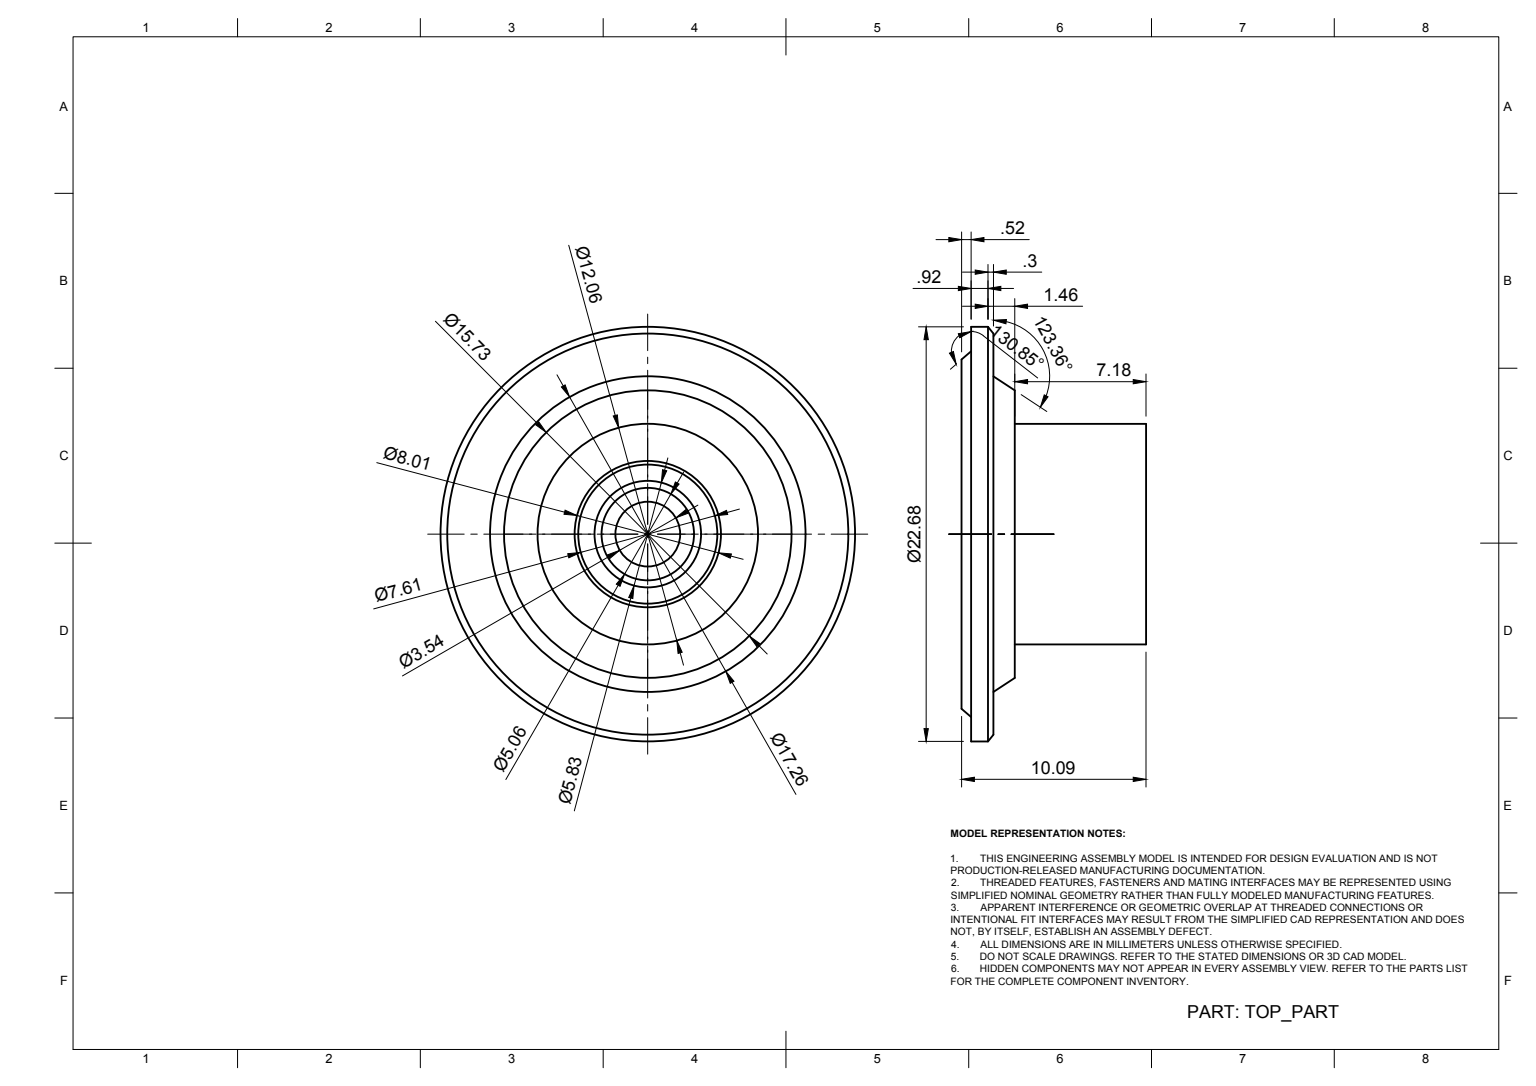
ISO-10303-21;
HEADER;
/* Generated by software containing ST-Developer
 * from STEP Tools, Inc. (www.steptools.com) 
 */

FILE_DESCRIPTION(
/* description */ (''),
/* implementation_level */ '2;1');

FILE_NAME(
/* name */ 'Top_Part.step',
/* time_stamp */ '2026-10-04T22:56:18-07:00',
/* author */ (''),
/* organization */ (''),
/* preprocessor_version */ 'ST-DEVELOPER v20.2',
/* originating_system */ 'Autodesk Translation Framework v15.15.0.0',
/* authorisation */ '');

FILE_SCHEMA (('AUTOMOTIVE_DESIGN { 1 0 10303 214 3 1 1 }'));
ENDSEC;

DATA;
#10=MECHANICAL_DESIGN_GEOMETRIC_PRESENTATION_REPRESENTATION('',(#196),#14544);
#44=CONICAL_SURFACE('',#2051,6.94221583892671,0.735432745767903);
#45=CONICAL_SURFACE('',#2055,9.77637943942299,0.712897062744303);
#46=CONICAL_SURFACE('',#2061,11.1537701181833,0.893668754257897);
#47=CONICAL_SURFACE('',#2065,8.2465180845384,0.582247271411204);
#48=CONICAL_SURFACE('',#2073,3.90337928524842,0.252845151189765);
#49=CONICAL_SURFACE('',#2083,2.14952775522097,1.03539162387167);
#180=SHAPE_REPRESENTATION_RELATIONSHIP('SRR','None',#14582,#188);
#188=ADVANCED_BREP_SHAPE_REPRESENTATION('',(#204),#14542);
#196=STYLED_ITEM('',(#14627),#204);
#204=MANIFOLD_SOLID_BREP('Body1',#1832);
#240=LINE('',#8609,#296);
#241=LINE('',#8617,#297);
#242=LINE('',#8624,#298);
#243=LINE('',#8627,#299);
#244=LINE('',#8634,#300);
#245=LINE('',#8642,#301);
#246=LINE('',#8649,#302);
#247=LINE('',#8656,#303);
#248=LINE('',#8663,#304);
#249=LINE('',#8667,#305);
#250=LINE('',#8669,#306);
#296=VECTOR('',#2420,6.94221583892671);
#297=VECTOR('',#2431,9.77637943942299);
#298=VECTOR('',#2440,11.3384150169577);
#299=VECTOR('',#2443,11.1537701181833);
#300=VECTOR('',#2452,8.2465180845384);
#301=VECTOR('',#2463,6.03157539652109);
#302=VECTOR('',#2472,3.90337928524842);
#303=VECTOR('',#2481,2.91473371720024);
#304=VECTOR('',#2490,2.52802020062926);
#305=VECTOR('',#2495,2.14952775522097);
#306=VECTOR('',#2498,1.77103530981268);
#353=CYLINDRICAL_SURFACE('',#2059,11.3384150169577);
#354=CYLINDRICAL_SURFACE('',#2069,6.03157539652109);
#355=CYLINDRICAL_SURFACE('',#2077,2.91473371720024);
#356=CYLINDRICAL_SURFACE('',#2081,2.52802020062926);
#357=CYLINDRICAL_SURFACE('',#2085,1.77103530981268);
#389=FACE_BOUND('',#589,.T.);
#390=FACE_BOUND('',#592,.T.);
#391=FACE_BOUND('',#595,.T.);
#392=FACE_BOUND('',#599,.T.);
#393=FACE_BOUND('',#602,.T.);
#394=FACE_BOUND('',#605,.T.);
#395=FACE_BOUND('',#608,.T.);
#396=FACE_BOUND('',#611,.T.);
#464=FACE_OUTER_BOUND('',#588,.T.);
#465=FACE_OUTER_BOUND('',#590,.T.);
#466=FACE_OUTER_BOUND('',#591,.T.);
#467=FACE_OUTER_BOUND('',#593,.T.);
#468=FACE_OUTER_BOUND('',#594,.T.);
#469=FACE_OUTER_BOUND('',#596,.T.);
#470=FACE_OUTER_BOUND('',#597,.T.);
#471=FACE_OUTER_BOUND('',#598,.T.);
#472=FACE_OUTER_BOUND('',#600,.T.);
#473=FACE_OUTER_BOUND('',#601,.T.);
#474=FACE_OUTER_BOUND('',#603,.T.);
#475=FACE_OUTER_BOUND('',#604,.T.);
#476=FACE_OUTER_BOUND('',#606,.T.);
#477=FACE_OUTER_BOUND('',#607,.T.);
#478=FACE_OUTER_BOUND('',#609,.T.);
#479=FACE_OUTER_BOUND('',#610,.T.);
#480=FACE_OUTER_BOUND('',#612,.T.);
#481=FACE_OUTER_BOUND('',#613,.T.);
#482=FACE_OUTER_BOUND('',#614,.T.);
#588=EDGE_LOOP('',(#1481));
#589=EDGE_LOOP('',(#1482));
#590=EDGE_LOOP('',(#1483,#1484,#1485,#1486));
#591=EDGE_LOOP('',(#1487));
#592=EDGE_LOOP('',(#1488));
#593=EDGE_LOOP('',(#1489,#1490,#1491,#1492));
#594=EDGE_LOOP('',(#1493));
#595=EDGE_LOOP('',(#1494));
#596=EDGE_LOOP('',(#1495,#1496,#1497,#1498));
#597=EDGE_LOOP('',(#1499,#1500,#1501,#1502));
#598=EDGE_LOOP('',(#1503));
#599=EDGE_LOOP('',(#1504));
#600=EDGE_LOOP('',(#1505,#1506,#1507,#1508));
#601=EDGE_LOOP('',(#1509));
#602=EDGE_LOOP('',(#1510));
#603=EDGE_LOOP('',(#1511,#1512,#1513,#1514));
#604=EDGE_LOOP('',(#1515));
#605=EDGE_LOOP('',(#1516));
#606=EDGE_LOOP('',(#1517,#1518,#1519,#1520));
#607=EDGE_LOOP('',(#1521));
#608=EDGE_LOOP('',(#1522));
#609=EDGE_LOOP('',(#1523,#1524,#1525,#1526));
#610=EDGE_LOOP('',(#1527));
#611=EDGE_LOOP('',(#1528));
#612=EDGE_LOOP('',(#1529,#1530,#1531,#1532));
#613=EDGE_LOOP('',(#1533,#1534,#1535,#1536));
#614=EDGE_LOOP('',(#1537,#1538,#1539,#1540));
#692=CIRCLE('',#2049,6.73223109314486);
#693=CIRCLE('',#2050,1.77103530981268);
#694=CIRCLE('',#2052,7.15220058470855);
#695=CIRCLE('',#2054,9.55065635544564);
#696=CIRCLE('',#2056,10.0021025234003);
#697=CIRCLE('',#2058,11.3384150169577);
#698=CIRCLE('',#2060,11.3384150169577);
#699=CIRCLE('',#2062,10.9691252194088);
#700=CIRCLE('',#2064,8.63028983493237);
#701=CIRCLE('',#2066,7.86274633414444);
#702=CIRCLE('',#2068,6.03157539652109);
#703=CIRCLE('',#2070,6.03157539652109);
#704=CIRCLE('',#2072,4.0030788546633);
#705=CIRCLE('',#2074,3.80367971583355);
#706=CIRCLE('',#2076,2.91473371720024);
#707=CIRCLE('',#2078,2.91473371720024);
#708=CIRCLE('',#2080,2.52802020062926);
#709=CIRCLE('',#2082,2.52802020062926);
#710=CIRCLE('',#2084,1.77103530981268);
#840=VERTEX_POINT('',#8603);
#841=VERTEX_POINT('',#8605);
#842=VERTEX_POINT('',#8608);
#843=VERTEX_POINT('',#8612);
#844=VERTEX_POINT('',#8615);
#845=VERTEX_POINT('',#8619);
#846=VERTEX_POINT('',#8622);
#847=VERTEX_POINT('',#8626);
#848=VERTEX_POINT('',#8630);
#849=VERTEX_POINT('',#8633);
#850=VERTEX_POINT('',#8637);
#851=VERTEX_POINT('',#8640);
#852=VERTEX_POINT('',#8644);
#853=VERTEX_POINT('',#8647);
#854=VERTEX_POINT('',#8651);
#855=VERTEX_POINT('',#8654);
#856=VERTEX_POINT('',#8658);
#857=VERTEX_POINT('',#8661);
#858=VERTEX_POINT('',#8665);
#1069=EDGE_CURVE('',#840,#840,#692,.T.);
#1070=EDGE_CURVE('',#841,#841,#693,.T.);
#1071=EDGE_CURVE('',#840,#842,#240,.T.);
#1072=EDGE_CURVE('',#842,#842,#694,.T.);
#1073=EDGE_CURVE('',#843,#843,#695,.T.);
#1074=EDGE_CURVE('',#844,#844,#696,.T.);
#1075=EDGE_CURVE('',#844,#843,#241,.T.);
#1076=EDGE_CURVE('',#845,#845,#697,.T.);
#1077=EDGE_CURVE('',#846,#846,#698,.T.);
#1078=EDGE_CURVE('',#846,#845,#242,.T.);
#1079=EDGE_CURVE('',#846,#847,#243,.T.);
#1080=EDGE_CURVE('',#847,#847,#699,.T.);
#1081=EDGE_CURVE('',#848,#848,#700,.T.);
#1082=EDGE_CURVE('',#848,#849,#244,.T.);
#1083=EDGE_CURVE('',#849,#849,#701,.T.);
#1084=EDGE_CURVE('',#850,#850,#702,.T.);
#1085=EDGE_CURVE('',#851,#851,#703,.T.);
#1086=EDGE_CURVE('',#851,#850,#245,.T.);
#1087=EDGE_CURVE('',#852,#852,#704,.T.);
#1088=EDGE_CURVE('',#853,#853,#705,.T.);
#1089=EDGE_CURVE('',#853,#852,#246,.T.);
#1090=EDGE_CURVE('',#854,#854,#706,.T.);
#1091=EDGE_CURVE('',#855,#855,#707,.T.);
#1092=EDGE_CURVE('',#855,#854,#247,.T.);
#1093=EDGE_CURVE('',#856,#856,#708,.T.);
#1094=EDGE_CURVE('',#857,#857,#709,.T.);
#1095=EDGE_CURVE('',#857,#856,#248,.T.);
#1096=EDGE_CURVE('',#858,#858,#710,.T.);
#1097=EDGE_CURVE('',#858,#857,#249,.T.);
#1098=EDGE_CURVE('',#841,#858,#250,.T.);
#1481=ORIENTED_EDGE('',*,*,#1069,.F.);
#1482=ORIENTED_EDGE('',*,*,#1070,.T.);
#1483=ORIENTED_EDGE('',*,*,#1069,.T.);
#1484=ORIENTED_EDGE('',*,*,#1071,.T.);
#1485=ORIENTED_EDGE('',*,*,#1072,.F.);
#1486=ORIENTED_EDGE('',*,*,#1071,.F.);
#1487=ORIENTED_EDGE('',*,*,#1073,.F.);
#1488=ORIENTED_EDGE('',*,*,#1072,.T.);
#1489=ORIENTED_EDGE('',*,*,#1074,.F.);
#1490=ORIENTED_EDGE('',*,*,#1075,.T.);
#1491=ORIENTED_EDGE('',*,*,#1073,.T.);
#1492=ORIENTED_EDGE('',*,*,#1075,.F.);
#1493=ORIENTED_EDGE('',*,*,#1076,.F.);
#1494=ORIENTED_EDGE('',*,*,#1074,.T.);
#1495=ORIENTED_EDGE('',*,*,#1077,.F.);
#1496=ORIENTED_EDGE('',*,*,#1078,.T.);
#1497=ORIENTED_EDGE('',*,*,#1076,.T.);
#1498=ORIENTED_EDGE('',*,*,#1078,.F.);
#1499=ORIENTED_EDGE('',*,*,#1077,.T.);
#1500=ORIENTED_EDGE('',*,*,#1079,.T.);
#1501=ORIENTED_EDGE('',*,*,#1080,.F.);
#1502=ORIENTED_EDGE('',*,*,#1079,.F.);
#1503=ORIENTED_EDGE('',*,*,#1080,.T.);
#1504=ORIENTED_EDGE('',*,*,#1081,.F.);
#1505=ORIENTED_EDGE('',*,*,#1081,.T.);
#1506=ORIENTED_EDGE('',*,*,#1082,.T.);
#1507=ORIENTED_EDGE('',*,*,#1083,.F.);
#1508=ORIENTED_EDGE('',*,*,#1082,.F.);
#1509=ORIENTED_EDGE('',*,*,#1083,.T.);
#1510=ORIENTED_EDGE('',*,*,#1084,.F.);
#1511=ORIENTED_EDGE('',*,*,#1085,.F.);
#1512=ORIENTED_EDGE('',*,*,#1086,.T.);
#1513=ORIENTED_EDGE('',*,*,#1084,.T.);
#1514=ORIENTED_EDGE('',*,*,#1086,.F.);
#1515=ORIENTED_EDGE('',*,*,#1085,.T.);
#1516=ORIENTED_EDGE('',*,*,#1087,.F.);
#1517=ORIENTED_EDGE('',*,*,#1088,.F.);
#1518=ORIENTED_EDGE('',*,*,#1089,.T.);
#1519=ORIENTED_EDGE('',*,*,#1087,.T.);
#1520=ORIENTED_EDGE('',*,*,#1089,.F.);
#1521=ORIENTED_EDGE('',*,*,#1088,.T.);
#1522=ORIENTED_EDGE('',*,*,#1090,.F.);
#1523=ORIENTED_EDGE('',*,*,#1091,.F.);
#1524=ORIENTED_EDGE('',*,*,#1092,.T.);
#1525=ORIENTED_EDGE('',*,*,#1090,.T.);
#1526=ORIENTED_EDGE('',*,*,#1092,.F.);
#1527=ORIENTED_EDGE('',*,*,#1091,.T.);
#1528=ORIENTED_EDGE('',*,*,#1093,.F.);
#1529=ORIENTED_EDGE('',*,*,#1094,.F.);
#1530=ORIENTED_EDGE('',*,*,#1095,.T.);
#1531=ORIENTED_EDGE('',*,*,#1093,.T.);
#1532=ORIENTED_EDGE('',*,*,#1095,.F.);
#1533=ORIENTED_EDGE('',*,*,#1096,.F.);
#1534=ORIENTED_EDGE('',*,*,#1097,.T.);
#1535=ORIENTED_EDGE('',*,*,#1094,.T.);
#1536=ORIENTED_EDGE('',*,*,#1097,.F.);
#1537=ORIENTED_EDGE('',*,*,#1070,.F.);
#1538=ORIENTED_EDGE('',*,*,#1098,.T.);
#1539=ORIENTED_EDGE('',*,*,#1096,.T.);
#1540=ORIENTED_EDGE('',*,*,#1098,.F.);
#1708=PLANE('',#2048);
#1709=PLANE('',#2053);
#1710=PLANE('',#2057);
#1711=PLANE('',#2063);
#1712=PLANE('',#2067);
#1713=PLANE('',#2071);
#1714=PLANE('',#2075);
#1715=PLANE('',#2079);
#1786=ADVANCED_FACE('',(#464,#389),#1708,.T.);
#1787=ADVANCED_FACE('',(#465),#44,.F.);
#1788=ADVANCED_FACE('',(#466,#390),#1709,.T.);
#1789=ADVANCED_FACE('',(#467),#45,.T.);
#1790=ADVANCED_FACE('',(#468,#391),#1710,.T.);
#1791=ADVANCED_FACE('',(#469),#353,.T.);
#1792=ADVANCED_FACE('',(#470),#46,.T.);
#1793=ADVANCED_FACE('',(#471,#392),#1711,.T.);
#1794=ADVANCED_FACE('',(#472),#47,.T.);
#1795=ADVANCED_FACE('',(#473,#393),#1712,.T.);
#1796=ADVANCED_FACE('',(#474),#354,.T.);
#1797=ADVANCED_FACE('',(#475,#394),#1713,.T.);
#1798=ADVANCED_FACE('',(#476),#48,.F.);
#1799=ADVANCED_FACE('',(#477,#395),#1714,.T.);
#1800=ADVANCED_FACE('',(#478),#355,.F.);
#1801=ADVANCED_FACE('',(#479,#396),#1715,.T.);
#1802=ADVANCED_FACE('',(#480),#356,.F.);
#1803=ADVANCED_FACE('',(#481),#49,.F.);
#1804=ADVANCED_FACE('',(#482),#357,.F.);
#1832=CLOSED_SHELL('',(#1786,#1787,#1788,#1789,#1790,#1791,#1792,#1793,
#1794,#1795,#1796,#1797,#1798,#1799,#1800,#1801,#1802,#1803,#1804));
#2047=AXIS2_PLACEMENT_3D('',#8601,#2410,#2411);
#2048=AXIS2_PLACEMENT_3D('',#8602,#2412,#2413);
#2049=AXIS2_PLACEMENT_3D('',#8604,#2414,#2415);
#2050=AXIS2_PLACEMENT_3D('',#8606,#2416,#2417);
#2051=AXIS2_PLACEMENT_3D('',#8607,#2418,#2419);
#2052=AXIS2_PLACEMENT_3D('',#8610,#2421,#2422);
#2053=AXIS2_PLACEMENT_3D('',#8611,#2423,#2424);
#2054=AXIS2_PLACEMENT_3D('',#8613,#2425,#2426);
#2055=AXIS2_PLACEMENT_3D('',#8614,#2427,#2428);
#2056=AXIS2_PLACEMENT_3D('',#8616,#2429,#2430);
#2057=AXIS2_PLACEMENT_3D('',#8618,#2432,#2433);
#2058=AXIS2_PLACEMENT_3D('',#8620,#2434,#2435);
#2059=AXIS2_PLACEMENT_3D('',#8621,#2436,#2437);
#2060=AXIS2_PLACEMENT_3D('',#8623,#2438,#2439);
#2061=AXIS2_PLACEMENT_3D('',#8625,#2441,#2442);
#2062=AXIS2_PLACEMENT_3D('',#8628,#2444,#2445);
#2063=AXIS2_PLACEMENT_3D('',#8629,#2446,#2447);
#2064=AXIS2_PLACEMENT_3D('',#8631,#2448,#2449);
#2065=AXIS2_PLACEMENT_3D('',#8632,#2450,#2451);
#2066=AXIS2_PLACEMENT_3D('',#8635,#2453,#2454);
#2067=AXIS2_PLACEMENT_3D('',#8636,#2455,#2456);
#2068=AXIS2_PLACEMENT_3D('',#8638,#2457,#2458);
#2069=AXIS2_PLACEMENT_3D('',#8639,#2459,#2460);
#2070=AXIS2_PLACEMENT_3D('',#8641,#2461,#2462);
#2071=AXIS2_PLACEMENT_3D('',#8643,#2464,#2465);
#2072=AXIS2_PLACEMENT_3D('',#8645,#2466,#2467);
#2073=AXIS2_PLACEMENT_3D('',#8646,#2468,#2469);
#2074=AXIS2_PLACEMENT_3D('',#8648,#2470,#2471);
#2075=AXIS2_PLACEMENT_3D('',#8650,#2473,#2474);
#2076=AXIS2_PLACEMENT_3D('',#8652,#2475,#2476);
#2077=AXIS2_PLACEMENT_3D('',#8653,#2477,#2478);
#2078=AXIS2_PLACEMENT_3D('',#8655,#2479,#2480);
#2079=AXIS2_PLACEMENT_3D('',#8657,#2482,#2483);
#2080=AXIS2_PLACEMENT_3D('',#8659,#2484,#2485);
#2081=AXIS2_PLACEMENT_3D('',#8660,#2486,#2487);
#2082=AXIS2_PLACEMENT_3D('',#8662,#2488,#2489);
#2083=AXIS2_PLACEMENT_3D('',#8664,#2491,#2492);
#2084=AXIS2_PLACEMENT_3D('',#8666,#2493,#2494);
#2085=AXIS2_PLACEMENT_3D('',#8668,#2496,#2497);
#2410=DIRECTION('axis',(0.,0.,1.));
#2411=DIRECTION('refdir',(1.,0.,0.));
#2412=DIRECTION('center_axis',(0.,0.,-1.));
#2413=DIRECTION('ref_axis',(-1.,0.,0.));
#2414=DIRECTION('center_axis',(0.,0.,1.));
#2415=DIRECTION('ref_axis',(1.,0.,0.));
#2416=DIRECTION('center_axis',(0.,0.,1.));
#2417=DIRECTION('ref_axis',(1.,0.,0.));
#2418=DIRECTION('center_axis',(0.,0.,-1.));
#2419=DIRECTION('ref_axis',(1.,0.,0.));
#2420=DIRECTION('',(-0.670908116956861,8.21625477953198E-17,-0.74154049019686));
#2421=DIRECTION('center_axis',(0.,0.,1.));
#2422=DIRECTION('ref_axis',(1.,0.,0.));
#2423=DIRECTION('center_axis',(0.,0.,-1.));
#2424=DIRECTION('ref_axis',(-1.,0.,0.));
#2425=DIRECTION('center_axis',(0.,0.,1.));
#2426=DIRECTION('ref_axis',(1.,0.,0.));
#2427=DIRECTION('center_axis',(0.,0.,1.));
#2428=DIRECTION('ref_axis',(1.,0.,0.));
#2429=DIRECTION('center_axis',(0.,0.,1.));
#2430=DIRECTION('ref_axis',(1.,0.,0.));
#2431=DIRECTION('',(0.654028054476354,8.00953363467037E-17,-0.756470292845579));
#2432=DIRECTION('center_axis',(0.,0.,-1.));
#2433=DIRECTION('ref_axis',(-1.,0.,0.));
#2434=DIRECTION('center_axis',(0.,0.,1.));
#2435=DIRECTION('ref_axis',(1.,0.,0.));
#2436=DIRECTION('center_axis',(0.,0.,1.));
#2437=DIRECTION('ref_axis',(1.,0.,0.));
#2438=DIRECTION('center_axis',(0.,0.,1.));
#2439=DIRECTION('ref_axis',(1.,0.,0.));
#2440=DIRECTION('',(0.,0.,-1.));
#2441=DIRECTION('center_axis',(0.,0.,-1.));
#2442=DIRECTION('ref_axis',(1.,0.,0.));
#2443=DIRECTION('',(0.77937567080628,-9.54459920586232E-17,0.626556911824666));
#2444=DIRECTION('center_axis',(0.,0.,1.));
#2445=DIRECTION('ref_axis',(1.,0.,0.));
#2446=DIRECTION('center_axis',(0.,0.,1.));
#2447=DIRECTION('ref_axis',(1.,0.,0.));
#2448=DIRECTION('center_axis',(0.,0.,1.));
#2449=DIRECTION('ref_axis',(1.,0.,0.));
#2450=DIRECTION('center_axis',(0.,0.,-1.));
#2451=DIRECTION('ref_axis',(1.,0.,0.));
#2452=DIRECTION('',(0.549902309986816,-6.7343610376909E-17,0.835228980262996));
#2453=DIRECTION('center_axis',(0.,0.,1.));
#2454=DIRECTION('ref_axis',(1.,0.,0.));
#2455=DIRECTION('center_axis',(0.,0.,1.));
#2456=DIRECTION('ref_axis',(1.,0.,0.));
#2457=DIRECTION('center_axis',(0.,0.,1.));
#2458=DIRECTION('ref_axis',(1.,0.,0.));
#2459=DIRECTION('center_axis',(0.,0.,1.));
#2460=DIRECTION('ref_axis',(1.,0.,0.));
#2461=DIRECTION('center_axis',(0.,0.,1.));
#2462=DIRECTION('ref_axis',(1.,0.,0.));
#2463=DIRECTION('',(0.,0.,-1.));
#2464=DIRECTION('center_axis',(0.,0.,1.));
#2465=DIRECTION('ref_axis',(1.,0.,0.));
#2466=DIRECTION('center_axis',(0.,0.,1.));
#2467=DIRECTION('ref_axis',(1.,0.,0.));
#2468=DIRECTION('center_axis',(0.,0.,1.));
#2469=DIRECTION('ref_axis',(1.,0.,0.));
#2470=DIRECTION('center_axis',(0.,0.,1.));
#2471=DIRECTION('ref_axis',(1.,0.,0.));
#2472=DIRECTION('',(-0.250159656512074,-3.06357222623313E-17,0.968204599376475));
#2473=DIRECTION('center_axis',(0.,0.,1.));
#2474=DIRECTION('ref_axis',(1.,0.,0.));
#2475=DIRECTION('center_axis',(0.,0.,1.));
#2476=DIRECTION('ref_axis',(1.,0.,0.));
#2477=DIRECTION('center_axis',(0.,0.,1.));
#2478=DIRECTION('ref_axis',(1.,0.,0.));
#2479=DIRECTION('center_axis',(0.,0.,1.));
#2480=DIRECTION('ref_axis',(1.,0.,0.));
#2481=DIRECTION('',(0.,0.,1.));
#2482=DIRECTION('center_axis',(0.,0.,1.));
#2483=DIRECTION('ref_axis',(1.,0.,0.));
#2484=DIRECTION('center_axis',(0.,0.,1.));
#2485=DIRECTION('ref_axis',(1.,0.,0.));
#2486=DIRECTION('center_axis',(0.,0.,1.));
#2487=DIRECTION('ref_axis',(1.,0.,0.));
#2488=DIRECTION('center_axis',(0.,0.,1.));
#2489=DIRECTION('ref_axis',(1.,0.,0.));
#2490=DIRECTION('',(0.,0.,1.));
#2491=DIRECTION('center_axis',(0.,0.,1.));
#2492=DIRECTION('ref_axis',(1.,0.,0.));
#2493=DIRECTION('center_axis',(0.,0.,1.));
#2494=DIRECTION('ref_axis',(1.,0.,0.));
#2495=DIRECTION('',(-0.860062224672037,-1.05327245051216E-16,0.510189150896202));
#2496=DIRECTION('center_axis',(0.,0.,1.));
#2497=DIRECTION('ref_axis',(1.,0.,0.));
#2498=DIRECTION('',(0.,0.,1.));
#8601=CARTESIAN_POINT('',(0.,0.,0.));
#8602=CARTESIAN_POINT('Origin',(6.73223109314486,0.,86.2971179986903));
#8603=CARTESIAN_POINT('',(-6.73223109314486,-8.24460525934014E-16,86.2971179986903));
#8604=CARTESIAN_POINT('Origin',(0.,0.,86.2971179986903));
#8605=CARTESIAN_POINT('',(-1.77103530981268,-2.16889272333904E-16,86.2971179986903));
#8606=CARTESIAN_POINT('Origin',(0.,0.,86.2971179986903));
#8607=CARTESIAN_POINT('Origin',(0.,0.,86.0650263196877));
#8608=CARTESIAN_POINT('',(-7.15220058470855,-8.75891955292316E-16,85.8329346406852));
#8609=CARTESIAN_POINT('',(-6.94221583892671,8.50176240613165E-16,86.0650263196877));
#8610=CARTESIAN_POINT('Origin',(0.,0.,85.8329346406852));
#8611=CARTESIAN_POINT('Origin',(9.55065635544564,0.,85.8329346406852));
#8612=CARTESIAN_POINT('',(-9.55065635544564,-1.16961807354528E-15,85.8329346406852));
#8613=CARTESIAN_POINT('Origin',(0.,0.,85.8329346406852));
#8614=CARTESIAN_POINT('Origin',(0.,0.,86.0940133608864));
#8615=CARTESIAN_POINT('',(-10.0021025234003,-1.22490428400259E-15,86.3550920810876));
#8616=CARTESIAN_POINT('Origin',(0.,0.,86.3550920810876));
#8617=CARTESIAN_POINT('',(-9.77637943942299,-1.19726117877394E-15,86.0940133608864));
#8618=CARTESIAN_POINT('Origin',(11.3384150169577,0.,86.3550920810876));
#8619=CARTESIAN_POINT('',(-11.3384150169577,-1.38855536579215E-15,86.3550920810876));
#8620=CARTESIAN_POINT('Origin',(0.,0.,86.3550920810876));
#8621=CARTESIAN_POINT('Origin',(0.,0.,86.8168854949443));
#8622=CARTESIAN_POINT('',(-11.3384150169577,-1.38855536579215E-15,87.278678908801));
#8623=CARTESIAN_POINT('Origin',(0.,0.,87.278678908801));
#8624=CARTESIAN_POINT('',(-11.3384150169577,-1.38855536579215E-15,86.8168854949443));
#8625=CARTESIAN_POINT('Origin',(0.,0.,87.4271189254628));
#8626=CARTESIAN_POINT('',(-10.9691252194088,-1.34333040893955E-15,87.5755589421246));
#8627=CARTESIAN_POINT('',(-11.1537701181833,1.36594288736586E-15,87.4271189254628));
#8628=CARTESIAN_POINT('Origin',(0.,0.,87.5755589421246));
#8629=CARTESIAN_POINT('Origin',(8.63028983493237,0.,87.5755589421246));
#8630=CARTESIAN_POINT('',(-8.63028983493237,-1.05690568220639E-15,87.5755589421246));
#8631=CARTESIAN_POINT('Origin',(0.,0.,87.5755589421246));
#8632=CARTESIAN_POINT('Origin',(0.,0.,88.1584575441381));
#8633=CARTESIAN_POINT('',(-7.86274633414444,-9.62908713061757E-16,88.7413561461516));
#8634=CARTESIAN_POINT('',(-8.2465180845384,1.00990719763407E-15,88.1584575441381));
#8635=CARTESIAN_POINT('Origin',(0.,0.,88.7413561461516));
#8636=CARTESIAN_POINT('Origin',(6.03157539652109,0.,88.7413561461516));
#8637=CARTESIAN_POINT('',(-6.03157539652109,-7.38654950316548E-16,88.7413561461516));
#8638=CARTESIAN_POINT('Origin',(0.,0.,88.7413561461516));
#8639=CARTESIAN_POINT('Origin',(0.,0.,92.3318522386825));
#8640=CARTESIAN_POINT('',(-6.03157539652109,-7.38654950316548E-16,95.9223483312135));
#8641=CARTESIAN_POINT('Origin',(0.,0.,95.9223483312135));
#8642=CARTESIAN_POINT('',(-6.03157539652109,-7.38654950316548E-16,92.3318522386825));
#8643=CARTESIAN_POINT('Origin',(4.0030788546633,0.,95.9223483312135));
#8644=CARTESIAN_POINT('',(-4.0030788546633,-4.90235770609787E-16,95.9223483312135));
#8645=CARTESIAN_POINT('Origin',(0.,0.,95.9223483312135));
#8646=CARTESIAN_POINT('Origin',(0.,0.,95.536476432406));
#8647=CARTESIAN_POINT('',(-3.80367971583355,-4.65816418897727E-16,95.1506045335986));
#8648=CARTESIAN_POINT('Origin',(0.,0.,95.1506045335986));
#8649=CARTESIAN_POINT('',(-3.90337928524842,-4.78026094753756E-16,95.536476432406));
#8650=CARTESIAN_POINT('Origin',(2.91473371720024,0.,95.1506045335986));
#8651=CARTESIAN_POINT('',(-2.91473371720024,-3.56951931713614E-16,95.1506045335986));
#8652=CARTESIAN_POINT('Origin',(0.,0.,95.1506045335986));
#8653=CARTESIAN_POINT('Origin',(0.,0.,93.4125396072643));
#8654=CARTESIAN_POINT('',(-2.91473371720024,-3.56951931713614E-16,91.6744746809301));
#8655=CARTESIAN_POINT('Origin',(0.,0.,91.6744746809301));
#8656=CARTESIAN_POINT('',(-2.91473371720024,-3.56951931713614E-16,93.4125396072643));
#8657=CARTESIAN_POINT('Origin',(2.52802020062926,0.,91.6744746809301));
#8658=CARTESIAN_POINT('',(-2.52802020062926,-3.09593184688047E-16,91.6744746809301));
#8659=CARTESIAN_POINT('Origin',(0.,0.,91.6744746809301));
#8660=CARTESIAN_POINT('Origin',(0.,0.,90.2007950732064));
#8661=CARTESIAN_POINT('',(-2.52802020062926,-3.09593184688047E-16,88.7271154654827));
#8662=CARTESIAN_POINT('Origin',(0.,0.,88.7271154654827));
#8663=CARTESIAN_POINT('',(-2.52802020062926,-3.09593184688047E-16,90.2007950732064));
#8664=CARTESIAN_POINT('Origin',(0.,0.,88.5025936415912));
#8665=CARTESIAN_POINT('',(-1.77103530981268,-2.16889272333904E-16,88.2780718176998));
#8666=CARTESIAN_POINT('Origin',(0.,0.,88.2780718176998));
#8667=CARTESIAN_POINT('',(-2.14952775522097,-2.63241228510976E-16,88.5025936415912));
#8668=CARTESIAN_POINT('Origin',(0.,0.,87.287594908195));
#8669=CARTESIAN_POINT('',(-1.77103530981268,-2.16889272333904E-16,87.287594908195));
#14532=UNCERTAINTY_MEASURE_WITH_UNIT(LENGTH_MEASURE(0.01),#14545,
'DISTANCE_ACCURACY_VALUE',
'Maximum model space distance between geometric entities at asserted c
onnectivities');
#14534=UNCERTAINTY_MEASURE_WITH_UNIT(LENGTH_MEASURE(0.01),#14545,
'DISTANCE_ACCURACY_VALUE',
'Maximum model space distance between geometric entities at asserted c
onnectivities');
#14542=(
GEOMETRIC_REPRESENTATION_CONTEXT(3)
GLOBAL_UNCERTAINTY_ASSIGNED_CONTEXT((#14532))
GLOBAL_UNIT_ASSIGNED_CONTEXT((#14545,#14547,#14548))
REPRESENTATION_CONTEXT('','3D')
);
#14544=(
GEOMETRIC_REPRESENTATION_CONTEXT(3)
GLOBAL_UNCERTAINTY_ASSIGNED_CONTEXT((#14534))
GLOBAL_UNIT_ASSIGNED_CONTEXT((#14545,#14547,#14548))
REPRESENTATION_CONTEXT('','3D')
);
#14545=(
LENGTH_UNIT()
NAMED_UNIT(*)
SI_UNIT(.MILLI.,.METRE.)
);
#14547=(
NAMED_UNIT(*)
PLANE_ANGLE_UNIT()
SI_UNIT($,.RADIAN.)
);
#14548=(
NAMED_UNIT(*)
SI_UNIT($,.STERADIAN.)
SOLID_ANGLE_UNIT()
);
#14556=SHAPE_DEFINITION_REPRESENTATION(#14565,#14582);
#14565=PRODUCT_DEFINITION_SHAPE('',$,#14592);
#14582=SHAPE_REPRESENTATION('',(#2047),#14542);
#14584=PRODUCT_DEFINITION_CONTEXT('part definition',#14613,'design');
#14592=PRODUCT_DEFINITION('Top_Part','Top_Part',#14601,#14584);
#14601=PRODUCT_DEFINITION_FORMATION('',$,#14622);
#14613=APPLICATION_CONTEXT(
'Core Data for Automotive Mechanical Design Process');
#14614=PRODUCT_CONTEXT('part definition',#14613,'mechanical');
#14622=PRODUCT('Top_Part','Top_Part',$,(#14614));
#14627=PRESENTATION_STYLE_ASSIGNMENT((#14631));
#14631=SURFACE_STYLE_USAGE(.BOTH.,#14635);
#14635=SURFACE_SIDE_STYLE('',(#14639));
#14639=SURFACE_STYLE_FILL_AREA(#14643);
#14643=FILL_AREA_STYLE('Opaque(203,203,203)',(#14647));
#14647=FILL_AREA_STYLE_COLOUR('Opaque(203,203,203)',#14651);
#14651=COLOUR_RGB('Opaque(203,203,203)', 0.31764706, 0.68627451, 0.89019608);
ENDSEC;
END-ISO-10303-21;
